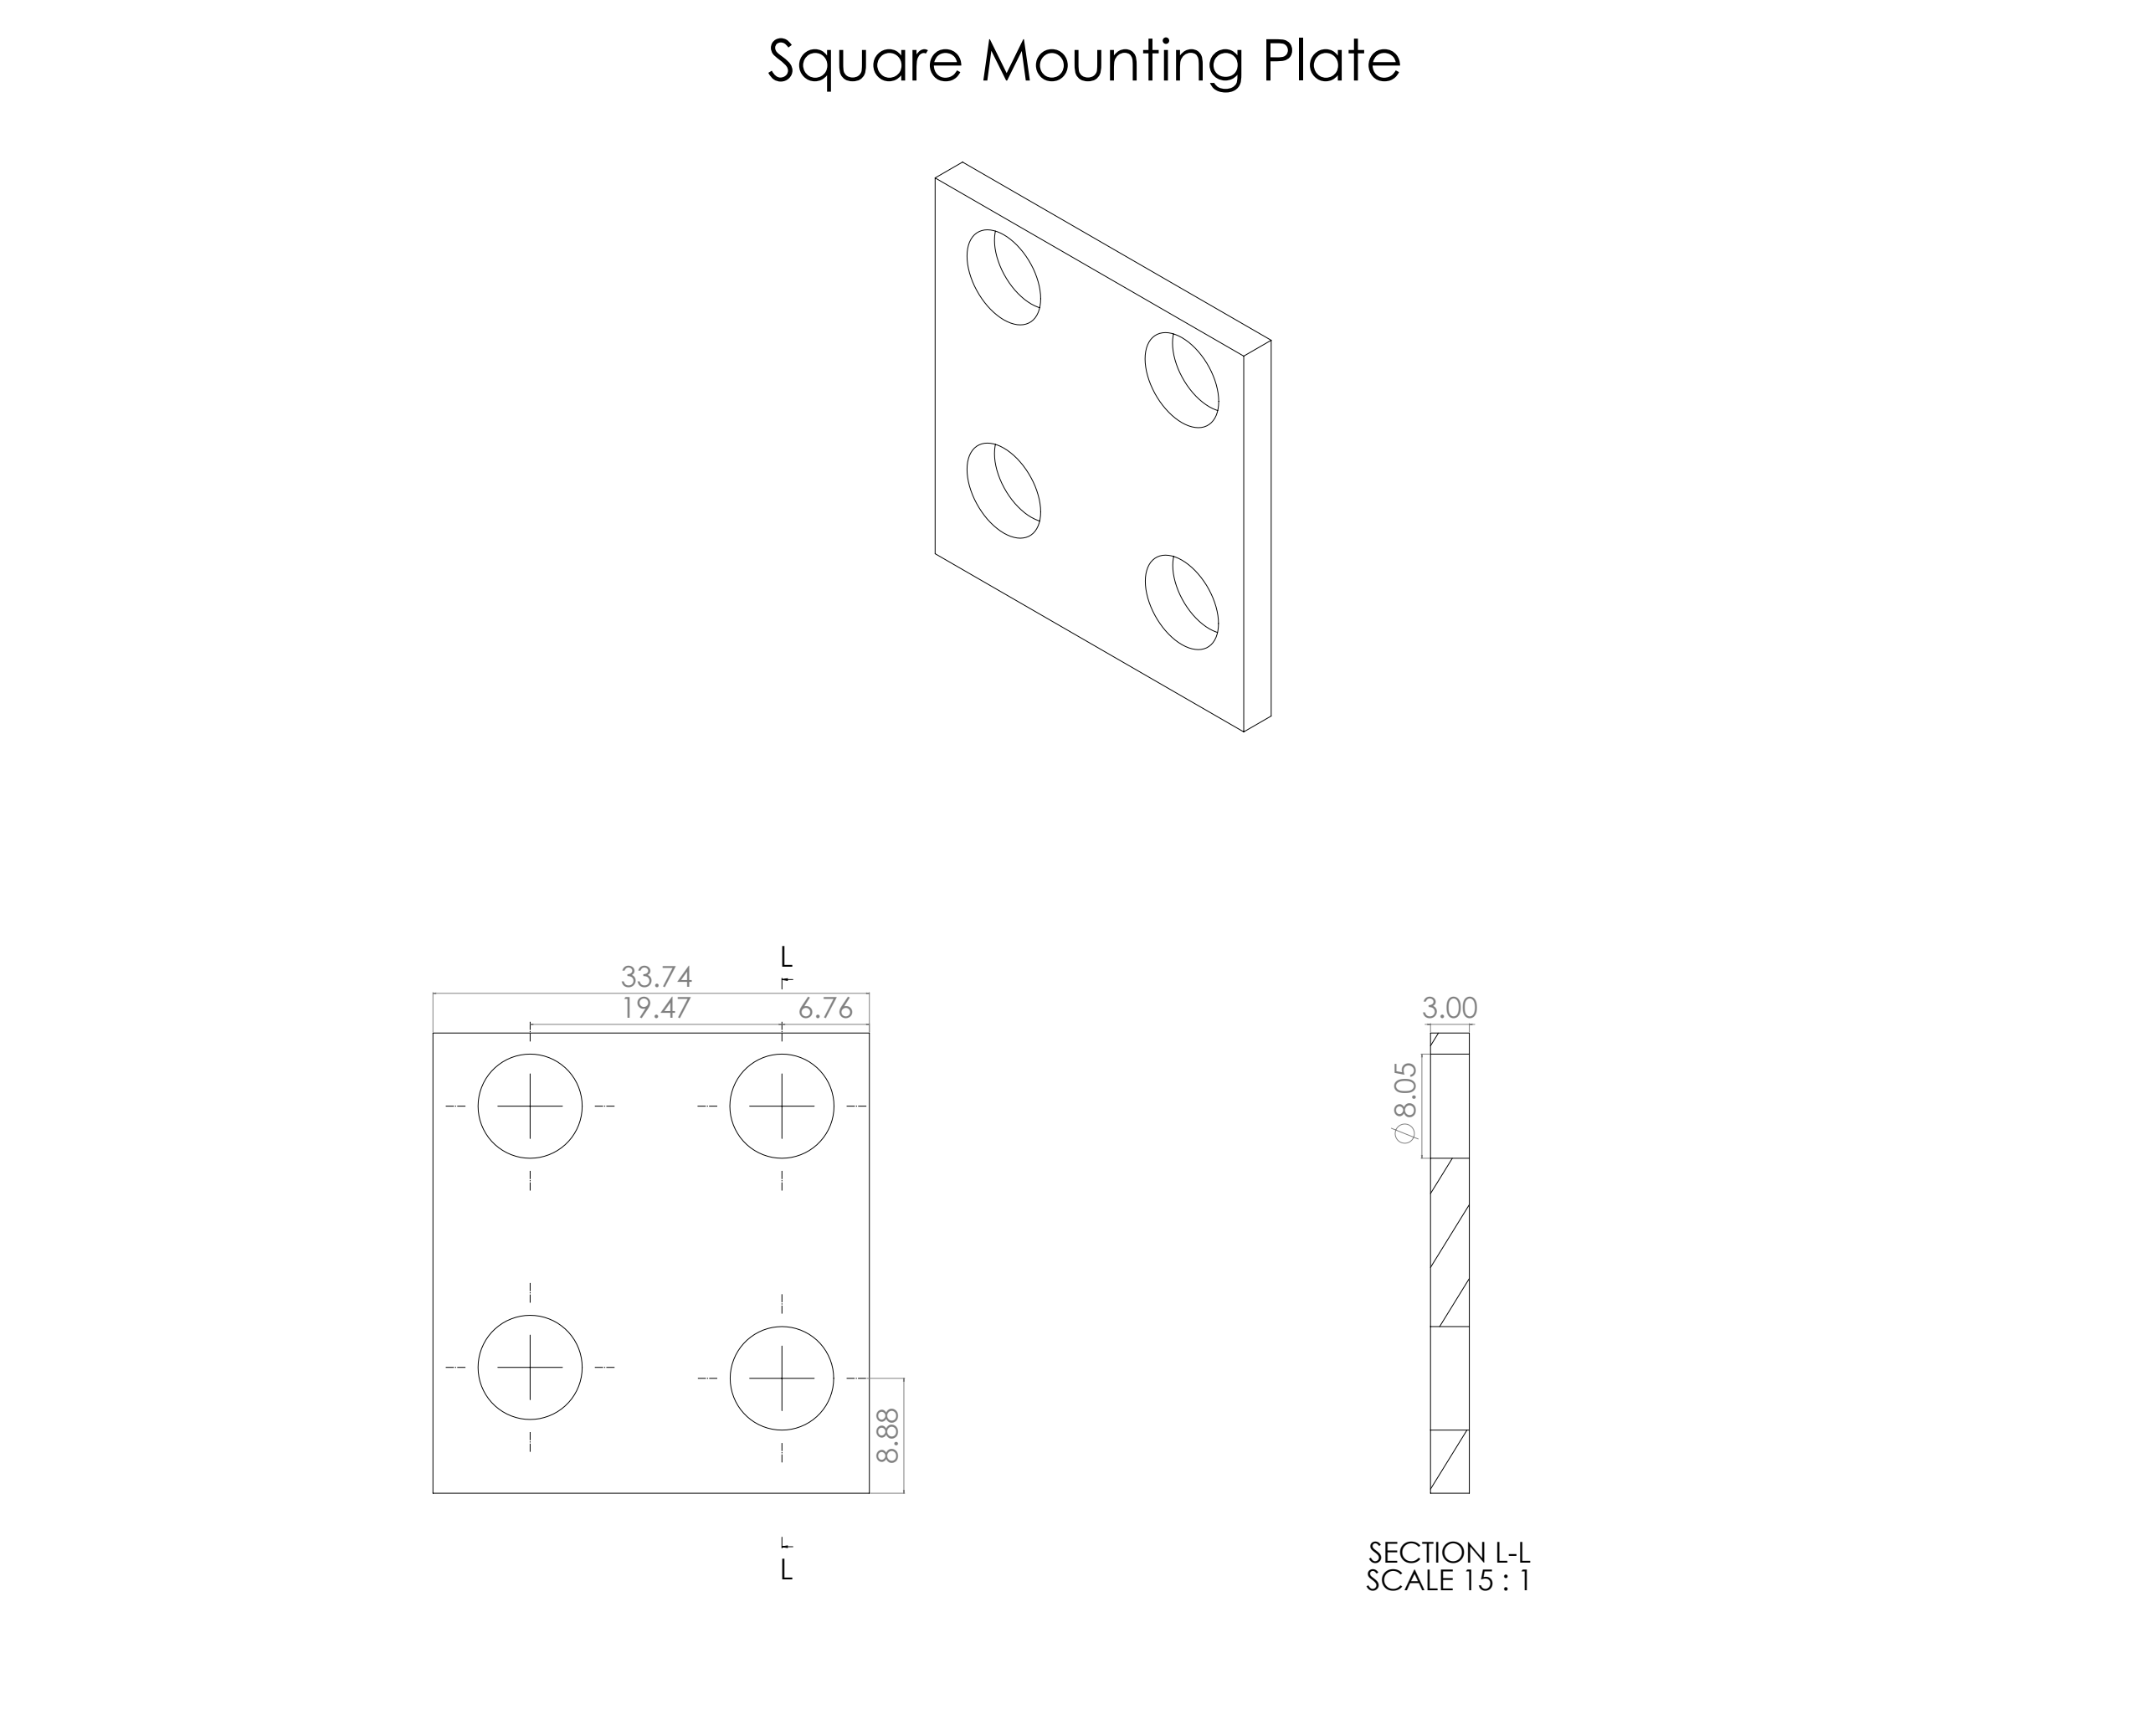
ISO-10303-21;
HEADER;
FILE_DESCRIPTION (('STEP AP214'),
    '1' );
FILE_NAME ('Square Mounting Plate.step',
    '2026-10-25T20:52:49',
    ( '' ),
    ( '' ),
    'SwSTEP 2.0',
    'SolidWorks 2025',
    '' );
FILE_SCHEMA (( 'AUTOMOTIVE_DESIGN' ));
ENDSEC;

DATA;
#8=AXIS2_PLACEMENT_3D ( 'NONE', #62573, #33196, #12356 ) ;
#139=DIRECTION ( 'NONE',  ( -0.000000000000000000, -0.000000000000000000, -1.000000000000000000 ) ) ;
#353=CARTESIAN_POINT ( 'NONE',  ( 184.7149167944524493, -12.49482340714361506, 10.00000000000000000 ) ) ;
#408=ORIENTED_EDGE ( 'NONE', *, *, #36940, .T. ) ;
#447=ADVANCED_FACE ( 'NONE', ( #62233, #49878, #84920, #20557, #27656 ), #19601, .F. ) ;
#551=CIRCLE ( 'NONE', #48930, 4.025000000000000355 ) ;
#864=UNCERTAINTY_MEASURE_WITH_UNIT (LENGTH_MEASURE( 1.000000000000000082E-05 ), #46095, 'distance_accuracy_value', 'NONE');
#1344=LINE ( 'NONE', #84136, #2329 ) ;
#1911=VERTEX_POINT ( 'NONE', #48237 ) ;
#1925=DIRECTION ( 'NONE',  ( 1.000000000000000000, 0.000000000000000000, 0.000000000000000000 ) ) ;
#2019=AXIS2_PLACEMENT_3D ( 'NONE', #11166, #32490, #12101 ) ;
#2104=VECTOR ( 'NONE', #19329, 1000.000000000000000 ) ;
#2329=VECTOR ( 'NONE', #75642, 1000.000000000000000 ) ;
#2393=ORIENTED_EDGE ( 'NONE', *, *, #76002, .F. ) ;
#2730=LINE ( 'NONE', #22180, #9659 ) ;
#2962=ORIENTED_EDGE ( 'NONE', *, *, #45806, .T. ) ;
#2974=ORIENTED_EDGE ( 'NONE', *, *, #32590, .F. ) ;
#3119=EDGE_CURVE ( 'NONE', #68047, #25647, #2730, .T. ) ;
#3129=PLANE ( 'NONE',  #2019 ) ;
#3367=ADVANCED_FACE ( 'NONE', ( #32552 ), #90725, .F. ) ;
#3593=DIRECTION ( 'NONE',  ( 0.000000000000000000, -1.000000000000000000, 0.000000000000000000 ) ) ;
#3609=DIRECTION ( 'NONE',  ( -0.000000000000000000, 1.000000000000000000, -0.000000000000000000 ) ) ;
#3701=ORIENTED_EDGE ( 'NONE', *, *, #20481, .F. ) ;
#4241=ORIENTED_EDGE ( 'NONE', *, *, #72732, .F. ) ;
#4407=CARTESIAN_POINT ( 'NONE',  ( 157.7374095173865385, 14.19731191252289015, 10.00000000000000000 ) ) ;
#4431=CARTESIAN_POINT ( 'NONE',  ( 157.7374095173865385, -21.37379927922774314, 13.00000000000000178 ) ) ;
#4459=CARTESIAN_POINT ( 'NONE',  ( 0.000000000000000000, 0.000000000000000000, 13.00000000000000178 ) ) ;
#4865=CARTESIAN_POINT ( 'NONE',  ( 165.2494399300530290, 8.542400036368780647, 13.00000000000000178 ) ) ;
#5292=AXIS2_PLACEMENT_3D ( 'NONE', #52984, #39682, #88956 ) ;
#5545=DIRECTION ( 'NONE',  ( -0.000000000000000000, -0.000000000000000000, -1.000000000000000000 ) ) ;
#5566=DIRECTION ( 'NONE',  ( 1.000000000000000000, 0.000000000000000000, 0.000000000000000000 ) ) ;
#5653=DIRECTION ( 'NONE',  ( 0.000000000000000000, 0.000000000000000000, 1.000000000000000000 ) ) ;
#5825=VECTOR ( 'NONE', #37864, 1000.000000000000000 ) ;
#6003=CYLINDRICAL_SURFACE ( 'NONE', #90095, 4.025000000000000355 ) ;
#6032=EDGE_CURVE ( 'NONE', #1911, #61737, #79312, .T. ) ;
#6390=CARTESIAN_POINT ( 'NONE',  ( 184.7149167944524493, 8.542400036368780647, 13.00000000000000178 ) ) ;
#6471=FACE_OUTER_BOUND ( 'NONE', #34561, .T. ) ;
#6537=DIRECTION ( 'NONE',  ( 0.000000000000000000, 0.000000000000000000, 1.000000000000000000 ) ) ;
#6539=CARTESIAN_POINT ( 'NONE',  ( 188.7399167944524550, 8.542400036368780647, 10.00000000000000000 ) ) ;
#6644=CIRCLE ( 'NONE', #42844, 4.025000000000000355 ) ;
#6791=ORIENTED_EDGE ( 'NONE', *, *, #15024, .T. ) ;
#6965=CARTESIAN_POINT ( 'NONE',  ( 184.7149167944524493, -12.49482340714361506, 13.00000000000000178 ) ) ;
#7630=DIRECTION ( 'NONE',  ( 0.000000000000000000, 0.000000000000000000, 1.000000000000000000 ) ) ;
#7706=ORIENTED_EDGE ( 'NONE', *, *, #10597, .T. ) ;
#7906=DIRECTION ( 'NONE',  ( 0.000000000000000000, -1.000000000000000000, 0.000000000000000000 ) ) ;
#8136=ADVANCED_FACE ( 'NONE', ( #24569 ), #18400, .F. ) ;
#8485=LINE ( 'NONE', #29817, #24717 ) ;
#8878=DIRECTION ( 'NONE',  ( 1.000000000000000000, 0.000000000000000000, 0.000000000000000000 ) ) ;
#9004=ORIENTED_EDGE ( 'NONE', *, *, #61815, .F. ) ;
#9377=PRODUCT_DEFINITION ( 'UNKNOWN', '', #37123, #92065 ) ;
#9659=VECTOR ( 'NONE', #77029, 1000.000000000000000 ) ;
#9802=DIRECTION ( 'NONE',  ( -1.000000000000000000, 0.000000000000000000, 0.000000000000000000 ) ) ;
#10162=ORIENTED_EDGE ( 'NONE', *, *, #76002, .T. ) ;
#10597=EDGE_CURVE ( 'NONE', #42154, #35472, #64044, .T. ) ;
#10869=SHAPE_DEFINITION_REPRESENTATION ( #16322, #67633 ) ;
#10909=ADVANCED_FACE ( 'NONE', ( #61387 ), #3129, .F. ) ;
#10927=DIRECTION ( 'NONE',  ( -0.000000000000000000, 1.000000000000000000, -0.000000000000000000 ) ) ;
#10938=ORIENTED_EDGE ( 'NONE', *, *, #71944, .T. ) ;
#11054=EDGE_CURVE ( 'NONE', #75279, #54193, #61836, .T. ) ;
#11126=ORIENTED_EDGE ( 'NONE', *, *, #61815, .T. ) ;
#11166=CARTESIAN_POINT ( 'NONE',  ( 191.4749582765727212, -21.37379927922774314, 13.00000000000000178 ) ) ;
#11214=ORIENTED_EDGE ( 'NONE', *, *, #3119, .F. ) ;
#11227=DIRECTION ( 'NONE',  ( -1.000000000000000000, 0.000000000000000000, 0.000000000000000000 ) ) ;
#11260=EDGE_CURVE ( 'NONE', #35472, #42154, #551, .T. ) ;
#12032=DIRECTION ( 'NONE',  ( -0.000000000000000000, 0.000000000000000000, -1.000000000000000000 ) ) ;
#12093=CARTESIAN_POINT ( 'NONE',  ( 157.7374095173865385, 14.19731191252289015, 13.00000000000000178 ) ) ;
#12101=DIRECTION ( 'NONE',  ( 0.000000000000000000, 0.000000000000000000, 1.000000000000000000 ) ) ;
#12158=DIRECTION ( 'NONE',  ( 0.000000000000000000, 0.000000000000000000, 1.000000000000000000 ) ) ;
#12159=CARTESIAN_POINT ( 'NONE',  ( 165.2494399300530290, -11.64849832608277325, 13.00000000000000178 ) ) ;
#12356=DIRECTION ( 'NONE',  ( 1.000000000000000000, 0.000000000000000000, 0.000000000000000000 ) ) ;
#12553=EDGE_CURVE ( 'NONE', #60279, #70988, #6644, .T. ) ;
#12633=VECTOR ( 'NONE', #3593, 1000.000000000000000 ) ;
#12712=CARTESIAN_POINT ( 'NONE',  ( 165.2494399300530290, 8.542400036368780647, 10.00000000000000000 ) ) ;
#12714=CARTESIAN_POINT ( 'NONE',  ( 161.2244399300530233, 8.542400036368780647, 13.00000000000000178 ) ) ;
#12853=ORIENTED_EDGE ( 'NONE', *, *, #17274, .F. ) ;
#13234=CARTESIAN_POINT ( 'NONE',  ( 157.7374095173865385, 14.19731191252289015, 13.00000000000000178 ) ) ;
#13610=DIRECTION ( 'NONE',  ( -0.000000000000000000, -0.000000000000000000, -1.000000000000000000 ) ) ;
#13683=VERTEX_POINT ( 'NONE', #44001 ) ;
#13955=ORIENTED_EDGE ( 'NONE', *, *, #89206, .T. ) ;
#13997=AXIS2_PLACEMENT_3D ( 'NONE', #6390, #21057, #20601 ) ;
#14168=CARTESIAN_POINT ( 'NONE',  ( 184.7149167944524493, 8.542400036368780647, 10.00000000000000000 ) ) ;
#14370=VERTEX_POINT ( 'NONE', #44472 ) ;
#15012=LINE ( 'NONE', #34924, #23160 ) ;
#15024=EDGE_CURVE ( 'NONE', #13683, #26669, #33933, .T. ) ;
#15028=DIRECTION ( 'NONE',  ( 0.000000000000000000, 0.000000000000000000, 1.000000000000000000 ) ) ;
#15052=CARTESIAN_POINT ( 'NONE',  ( 165.2494399300530290, -11.64849832608277325, 13.00000000000000178 ) ) ;
#15135=LINE ( 'NONE', #48894, #73055 ) ;
#15206=AXIS2_PLACEMENT_3D ( 'NONE', #88270, #45167, #75471 ) ;
#15346=( GEOMETRIC_REPRESENTATION_CONTEXT ( 3 ) GLOBAL_UNCERTAINTY_ASSIGNED_CONTEXT ( ( #864 ) ) GLOBAL_UNIT_ASSIGNED_CONTEXT ( ( #46095, #75000, #22926 ) ) REPRESENTATION_CONTEXT ( 'NONE', 'WORKASPACE' ) );
#15365=CYLINDRICAL_SURFACE ( 'NONE', #84868, 4.000000000000003553 ) ;
#15479=DIRECTION ( 'NONE',  ( 1.000000000000000000, 0.000000000000000000, 0.000000000000000000 ) ) ;
#15510=DIRECTION ( 'NONE',  ( -0.000000000000000000, -0.000000000000000000, -1.000000000000000000 ) ) ;
#15530=AXIS2_PLACEMENT_3D ( 'NONE', #4865, #91002, #77306 ) ;
#15570=VECTOR ( 'NONE', #139, 1000.000000000000000 ) ;
#15605=AXIS2_PLACEMENT_3D ( 'NONE', #59729, #88571, #45946 ) ;
#15644=EDGE_CURVE ( 'NONE', #54449, #93705, #66778, .T. ) ;
#16173=EDGE_CURVE ( 'NONE', #25647, #60166, #23043, .T. ) ;
#16322=PRODUCT_DEFINITION_SHAPE ( 'NONE', 'NONE',  #9377 ) ;
#16414=CARTESIAN_POINT ( 'NONE',  ( 157.7374095173865385, 14.19731191252289015, 10.00000000000000000 ) ) ;
#16631=DIRECTION ( 'NONE',  ( 0.000000000000000000, 0.000000000000000000, 1.000000000000000000 ) ) ;
#16908=CARTESIAN_POINT ( 'NONE',  ( 191.4749582765727212, -21.37379927922774314, 10.00000000000000000 ) ) ;
#16910=DIRECTION ( 'NONE',  ( 1.000000000000000000, 0.000000000000000000, 0.000000000000000000 ) ) ;
#17031=AXIS2_PLACEMENT_3D ( 'NONE', #6965, #37671, #45697 ) ;
#17057=PRODUCT_CONTEXT ( 'NONE', #52342, 'mechanical' ) ;
#17230=APPLICATION_CONTEXT ( 'automotive_design' ) ;
#17233=FACE_OUTER_BOUND ( 'NONE', #64373, .T. ) ;
#17274=EDGE_CURVE ( 'NONE', #75279, #79924, #47612, .T. ) ;
#17796=PLANE ( 'NONE',  #80542 ) ;
#17808=CARTESIAN_POINT ( 'NONE',  ( 165.2494399300530290, 8.542400036368780647, 13.00000000000000178 ) ) ;
#18181=EDGE_LOOP ( 'NONE', ( #55024, #55045, #4241, #85295 ) ) ;
#18204=EDGE_CURVE ( 'NONE', #60166, #54193, #90447, .T. ) ;
#18373=STYLED_ITEM('',(#93738),#58100);
#18377=CARTESIAN_POINT ( 'NONE',  ( 161.2244399300530233, 8.542400036368780647, 13.00000000000000178 ) ) ;
#18400=CYLINDRICAL_SURFACE ( 'NONE', #5292, 4.025000000000000355 ) ;
#18683=ORIENTED_EDGE ( 'NONE', *, *, #91573, .F. ) ;
#18731=FACE_BOUND ( 'NONE', #71920, .T. ) ;
#18940=AXIS2_PLACEMENT_3D ( 'NONE', #90959, #40773, #33703 ) ;
#19058=VERTEX_POINT ( 'NONE', #55447 ) ;
#19329=DIRECTION ( 'NONE',  ( -0.000000000000000000, -0.000000000000000000, -1.000000000000000000 ) ) ;
#19436=DIRECTION ( 'NONE',  ( -0.000000000000000000, -0.000000000000000000, -1.000000000000000000 ) ) ;
#19601=PLANE ( 'NONE',  #64162 ) ;
#19841=DIRECTION ( 'NONE',  ( -0.000000000000000000, 0.000000000000000000, -1.000000000000000000 ) ) ;
#20063=AXIS2_PLACEMENT_3D ( 'NONE', #71362, #56703, #5566 ) ;
#20449=CLOSED_SHELL ( 'NONE', ( #27401, #8136, #58097, #83433, #447, #23737, #3367, #41920, #88676, #10909, #93028, #88549, #21965, #23016 ) ) ;
#20454=ORIENTED_EDGE ( 'NONE', *, *, #88734, .F. ) ;
#20481=EDGE_CURVE ( 'NONE', #26669, #13683, #83518, .T. ) ;
#20511=CARTESIAN_POINT ( 'NONE',  ( 191.4749582765727212, -21.37379927922774314, 13.00000000000000178 ) ) ;
#20557=FACE_BOUND ( 'NONE', #43970, .T. ) ;
#20601=DIRECTION ( 'NONE',  ( -1.000000000000000000, 0.000000000000000000, 0.000000000000000000 ) ) ;
#21057=DIRECTION ( 'NONE',  ( -0.000000000000000000, -0.000000000000000000, -1.000000000000000000 ) ) ;
#21296=CIRCLE ( 'NONE', #15206, 4.025000000000000355 ) ;
#21478=ORIENTED_EDGE ( 'NONE', *, *, #26156, .F. ) ;
#21481=EDGE_LOOP ( 'NONE', ( #73742, #54532, #408, #40993 ) ) ;
#21520=FACE_OUTER_BOUND ( 'NONE', #59218, .T. ) ;
#21649=VECTOR ( 'NONE', #25477, 1000.000000000000000 ) ;
#21965=ADVANCED_FACE ( 'NONE', ( #21520 ), #73117, .F. ) ;
#22003=CIRCLE ( 'NONE', #56760, 4.025000000000000355 ) ;
#22180=CARTESIAN_POINT ( 'NONE',  ( 157.7374095173865385, 14.19731191252289015, 13.00000000000000178 ) ) ;
#22629=DIRECTION ( 'NONE',  ( 0.000000000000000000, 0.000000000000000000, 1.000000000000000000 ) ) ;
#22699=VECTOR ( 'NONE', #43051, 1000.000000000000000 ) ;
#22926=( NAMED_UNIT ( * ) SI_UNIT ( $, .STERADIAN. ) SOLID_ANGLE_UNIT ( ) );
#23016=ADVANCED_FACE ( 'NONE', ( #77785 ), #48403, .F. ) ;
#23025=CIRCLE ( 'NONE', #79013, 4.025000000000000355 ) ;
#23029=VECTOR ( 'NONE', #40726, 1000.000000000000000 ) ;
#23043=LINE ( 'NONE', #16414, #63840 ) ;
#23160=VECTOR ( 'NONE', #56730, 1000.000000000000000 ) ;
#23554=FACE_OUTER_BOUND ( 'NONE', #33852, .T. ) ;
#23680=CARTESIAN_POINT ( 'NONE',  ( 161.2244399300530233, -11.64849832608277325, 13.00000000000000178 ) ) ;
#23737=ADVANCED_FACE ( 'NONE', ( #18731, #41416, #47592, #55191, #68451 ), #17796, .T. ) ;
#23972=DIRECTION ( 'NONE',  ( 0.000000000000000000, 0.000000000000000000, 1.000000000000000000 ) ) ;
#24007=DIRECTION ( 'NONE',  ( 0.000000000000000000, 0.000000000000000000, 1.000000000000000000 ) ) ;
#24051=DIRECTION ( 'NONE',  ( 0.000000000000000000, 0.000000000000000000, 1.000000000000000000 ) ) ;
#24063=ORIENTED_EDGE ( 'NONE', *, *, #83965, .F. ) ;
#24181=CARTESIAN_POINT ( 'NONE',  ( 191.4749582765727212, 14.19731191252289015, 13.00000000000000178 ) ) ;
#24569=FACE_OUTER_BOUND ( 'NONE', #90079, .T. ) ;
#24717=VECTOR ( 'NONE', #77795, 1000.000000000000000 ) ;
#24915=CARTESIAN_POINT ( 'NONE',  ( 191.4749582765727212, -21.37379927922774314, 13.00000000000000178 ) ) ;
#25102=ORIENTED_EDGE ( 'NONE', *, *, #11054, .F. ) ;
#25477=DIRECTION ( 'NONE',  ( -0.000000000000000000, -0.000000000000000000, -1.000000000000000000 ) ) ;
#25493=LINE ( 'NONE', #12714, #2104 ) ;
#25592=LINE ( 'NONE', #54475, #91229 ) ;
#25647=VERTEX_POINT ( 'NONE', #4407 ) ;
#26156=EDGE_CURVE ( 'NONE', #78471, #75279, #15135, .T. ) ;
#26218=PRODUCT ( 'Square Mounting Plate', 'Square Mounting Plate', '', ( #17057 ) ) ;
#26330=EDGE_CURVE ( 'NONE', #79924, #68047, #8485, .T. ) ;
#26438=DIRECTION ( 'NONE',  ( 1.000000000000000000, 0.000000000000000000, 0.000000000000000000 ) ) ;
#26669=VERTEX_POINT ( 'NONE', #31668 ) ;
#27401=ADVANCED_FACE ( 'NONE', ( #82659 ), #52386, .F. ) ;
#27656=FACE_BOUND ( 'NONE', #56348, .T. ) ;
#27692=EDGE_LOOP ( 'NONE', ( #13955, #11214, #57944, #32676 ) ) ;
#27825=LINE ( 'NONE', #35844, #56523 ) ;
#27840=CARTESIAN_POINT ( 'NONE',  ( 161.2244399300530233, -11.64849832608277325, 10.00000000000000000 ) ) ;
#28163=CIRCLE ( 'NONE', #62975, 4.025000000000000355 ) ;
#28563=ORIENTED_EDGE ( 'NONE', *, *, #18204, .F. ) ;
#29388=EDGE_CURVE ( 'NONE', #54193, #19058, #75803, .T. ) ;
#29408=AXIS2_PLACEMENT_3D ( 'NONE', #90791, #62914, #26438 ) ;
#29498=ADVANCED_BREP_SHAPE_REPRESENTATION ( '', ( #58100, #18940 ), #56754 ) ;
#29762=ORIENTED_EDGE ( 'NONE', *, *, #26156, .T. ) ;
#29817=CARTESIAN_POINT ( 'NONE',  ( 191.4749582765727212, 14.19731191252289015, 13.00000000000000178 ) ) ;
#30553=ORIENTED_EDGE ( 'NONE', *, *, #18204, .T. ) ;
#30984=DIRECTION ( 'NONE',  ( -1.000000000000000000, 0.000000000000000000, 0.000000000000000000 ) ) ;
#31024=CARTESIAN_POINT ( 'NONE',  ( 161.2244399300530233, 8.542400036368780647, 10.00000000000000000 ) ) ;
#31087=DIRECTION ( 'NONE',  ( -0.000000000000000000, -0.000000000000000000, -1.000000000000000000 ) ) ;
#31668=CARTESIAN_POINT ( 'NONE',  ( 188.7149167944524493, -12.49482340714361506, 13.00000000000000178 ) ) ;
#32179=LINE ( 'NONE', #66768, #5825 ) ;
#32490=DIRECTION ( 'NONE',  ( 0.000000000000000000, 1.000000000000000000, -0.000000000000000000 ) ) ;
#32552=FACE_OUTER_BOUND ( 'NONE', #87279, .T. ) ;
#32590=EDGE_CURVE ( 'NONE', #79924, #19058, #57410, .T. ) ;
#32601=CARTESIAN_POINT ( 'NONE',  ( 191.4749582765727212, 14.19731191252289015, 13.00000000000000178 ) ) ;
#32676=ORIENTED_EDGE ( 'NONE', *, *, #32590, .T. ) ;
#33196=DIRECTION ( 'NONE',  ( 0.000000000000000000, 0.000000000000000000, 1.000000000000000000 ) ) ;
#33237=ORIENTED_EDGE ( 'NONE', *, *, #88734, .T. ) ;
#33703=DIRECTION ( 'NONE',  ( 1.000000000000000000, 0.000000000000000000, 0.000000000000000000 ) ) ;
#33711=CIRCLE ( 'NONE', #20063, 4.025000000000000355 ) ;
#33852=EDGE_LOOP ( 'NONE', ( #55744, #55923, #54648, #81093 ) ) ;
#33933=CIRCLE ( 'NONE', #29408, 4.000000000000003553 ) ;
#33939=AXIS2_PLACEMENT_3D ( 'NONE', #353, #15028, #43887 ) ;
#34528=FACE_OUTER_BOUND ( 'NONE', #21481, .T. ) ;
#34561=EDGE_LOOP ( 'NONE', ( #41948, #48478, #58414, #44534 ) ) ;
#34726=ORIENTED_EDGE ( 'NONE', *, *, #39657, .T. ) ;
#34779=ORIENTED_EDGE ( 'NONE', *, *, #51522, .T. ) ;
#34924=CARTESIAN_POINT ( 'NONE',  ( 169.2744399300530347, 8.542400036368780647, 13.00000000000000178 ) ) ;
#35006=LINE ( 'NONE', #77637, #22699 ) ;
#35018=AXIS2_PLACEMENT_3D ( 'NONE', #12712, #6537, #65245 ) ;
#35472=VERTEX_POINT ( 'NONE', #48415 ) ;
#35844=CARTESIAN_POINT ( 'NONE',  ( 180.6899167944524436, 8.542400036368780647, 13.00000000000000178 ) ) ;
#36042=EDGE_LOOP ( 'NONE', ( #34779, #43065, #77126, #64284 ) ) ;
#36581=LINE ( 'NONE', #71190, #15570 ) ;
#36781=CARTESIAN_POINT ( 'NONE',  ( 157.7374095173865385, -21.37379927922774314, 13.00000000000000178 ) ) ;
#36863=AXIS2_PLACEMENT_3D ( 'NONE', #88858, #24007, #16910 ) ;
#36940=EDGE_CURVE ( 'NONE', #13683, #61737, #25592, .T. ) ;
#37123=PRODUCT_DEFINITION_FORMATION_WITH_SPECIFIED_SOURCE ( 'ANY', '', #26218, .NOT_KNOWN. ) ;
#37671=DIRECTION ( 'NONE',  ( 0.000000000000000000, 0.000000000000000000, 1.000000000000000000 ) ) ;
#37864=DIRECTION ( 'NONE',  ( -0.000000000000000000, -0.000000000000000000, -1.000000000000000000 ) ) ;
#38735=EDGE_CURVE ( 'NONE', #70988, #54449, #25493, .T. ) ;
#39273=VERTEX_POINT ( 'NONE', #6539 ) ;
#39656=PLANE ( 'NONE',  #70119 ) ;
#39657=EDGE_CURVE ( 'NONE', #61737, #1911, #86848, .T. ) ;
#39682=DIRECTION ( 'NONE',  ( -0.000000000000000000, -0.000000000000000000, -1.000000000000000000 ) ) ;
#39846=CARTESIAN_POINT ( 'NONE',  ( 169.2744399300530347, 8.542400036368780647, 10.00000000000000000 ) ) ;
#40592=DIRECTION ( 'NONE',  ( 0.000000000000000000, -1.000000000000000000, 0.000000000000000000 ) ) ;
#40726=DIRECTION ( 'NONE',  ( 1.000000000000000000, -0.000000000000000000, -0.000000000000000000 ) ) ;
#40773=DIRECTION ( 'NONE',  ( 0.000000000000000000, 0.000000000000000000, 1.000000000000000000 ) ) ;
#40993=ORIENTED_EDGE ( 'NONE', *, *, #6032, .F. ) ;
#41416=FACE_BOUND ( 'NONE', #43459, .T. ) ;
#41475=ORIENTED_EDGE ( 'NONE', *, *, #89206, .F. ) ;
#41567=EDGE_CURVE ( 'NONE', #45901, #42154, #90323, .T. ) ;
#41920=ADVANCED_FACE ( 'NONE', ( #62900 ), #39656, .F. ) ;
#41948=ORIENTED_EDGE ( 'NONE', *, *, #78922, .F. ) ;
#42154=VERTEX_POINT ( 'NONE', #27840 ) ;
#42562=MECHANICAL_DESIGN_GEOMETRIC_PRESENTATION_REPRESENTATION('',(#18373),#15346);
#42844=AXIS2_PLACEMENT_3D ( 'NONE', #53556, #16631, #89983 ) ;
#43051=DIRECTION ( 'NONE',  ( -0.000000000000000000, -0.000000000000000000, -1.000000000000000000 ) ) ;
#43065=ORIENTED_EDGE ( 'NONE', *, *, #71361, .T. ) ;
#43288=EDGE_LOOP ( 'NONE', ( #54099, #11126 ) ) ;
#43459=EDGE_LOOP ( 'NONE', ( #7706, #69578 ) ) ;
#43871=LINE ( 'NONE', #36781, #54989 ) ;
#43887=DIRECTION ( 'NONE',  ( 1.000000000000000000, 0.000000000000000000, 0.000000000000000000 ) ) ;
#43970=EDGE_LOOP ( 'NONE', ( #73348, #67827 ) ) ;
#43998=DIRECTION ( 'NONE',  ( 1.000000000000000000, -0.000000000000000000, -0.000000000000000000 ) ) ;
#44001=CARTESIAN_POINT ( 'NONE',  ( 180.7149167944524493, -12.49482340714361506, 13.00000000000000178 ) ) ;
#44128=VERTEX_POINT ( 'NONE', #49507 ) ;
#44472=CARTESIAN_POINT ( 'NONE',  ( 188.7399167944524550, 8.542400036368780647, 13.00000000000000178 ) ) ;
#44534=ORIENTED_EDGE ( 'NONE', *, *, #11260, .F. ) ;
#45167=DIRECTION ( 'NONE',  ( 0.000000000000000000, 0.000000000000000000, 1.000000000000000000 ) ) ;
#45353=ORIENTED_EDGE ( 'NONE', *, *, #91573, .T. ) ;
#45697=DIRECTION ( 'NONE',  ( 1.000000000000000000, 0.000000000000000000, 0.000000000000000000 ) ) ;
#45768=CYLINDRICAL_SURFACE ( 'NONE', #61072, 4.025000000000000355 ) ;
#45806=EDGE_CURVE ( 'NONE', #26669, #1911, #32179, .T. ) ;
#45901=VERTEX_POINT ( 'NONE', #23680 ) ;
#45917=ORIENTED_EDGE ( 'NONE', *, *, #62258, .T. ) ;
#45946=DIRECTION ( 'NONE',  ( 1.000000000000000000, 0.000000000000000000, 0.000000000000000000 ) ) ;
#46095=( LENGTH_UNIT ( ) NAMED_UNIT ( * ) SI_UNIT ( .MILLI., .METRE. ) );
#46335=CARTESIAN_POINT ( 'NONE',  ( 157.7374095173865385, -21.37379927922774314, 10.00000000000000000 ) ) ;
#46649=DIRECTION ( 'NONE',  ( -1.000000000000000000, 0.000000000000000000, 0.000000000000000000 ) ) ;
#46661=DIRECTION ( 'NONE',  ( -0.000000000000000000, -0.000000000000000000, -1.000000000000000000 ) ) ;
#46696=ORIENTED_EDGE ( 'NONE', *, *, #29388, .F. ) ;
#47592=FACE_OUTER_BOUND ( 'NONE', #54104, .T. ) ;
#47612=LINE ( 'NONE', #68005, #85014 ) ;
#47652=AXIS2_PLACEMENT_3D ( 'NONE', #49197, #84694, #70528 ) ;
#48060=LINE ( 'NONE', #12093, #12633 ) ;
#48237=CARTESIAN_POINT ( 'NONE',  ( 188.7149167944524493, -12.49482340714361506, 10.00000000000000000 ) ) ;
#48403=CYLINDRICAL_SURFACE ( 'NONE', #15530, 4.025000000000000355 ) ;
#48415=CARTESIAN_POINT ( 'NONE',  ( 169.2744399300530347, -11.64849832608277325, 10.00000000000000000 ) ) ;
#48478=ORIENTED_EDGE ( 'NONE', *, *, #77975, .T. ) ;
#48894=CARTESIAN_POINT ( 'NONE',  ( 191.4749582765727212, -21.37379927922774314, 13.00000000000000178 ) ) ;
#48930=AXIS2_PLACEMENT_3D ( 'NONE', #63734, #58013, #72220 ) ;
#49017=VECTOR ( 'NONE', #53544, 1000.000000000000000 ) ;
#49171=EDGE_LOOP ( 'NONE', ( #34726, #73801 ) ) ;
#49197=CARTESIAN_POINT ( 'NONE',  ( 184.7149167944524493, -12.49482340714361506, 13.00000000000000178 ) ) ;
#49507=CARTESIAN_POINT ( 'NONE',  ( 180.6899167944524436, 8.542400036368780647, 13.00000000000000178 ) ) ;
#49644=EDGE_LOOP ( 'NONE', ( #30553, #25102, #21478, #10938 ) ) ;
#49878=FACE_BOUND ( 'NONE', #52581, .T. ) ;
#51413=CIRCLE ( 'NONE', #8, 4.025000000000000355 ) ;
#51522=EDGE_CURVE ( 'NONE', #70988, #60279, #51413, .T. ) ;
#51626=( NAMED_UNIT ( * ) PLANE_ANGLE_UNIT ( ) SI_UNIT ( $, .RADIAN. ) );
#52342=APPLICATION_CONTEXT ( 'automotive_design' ) ;
#52386=CYLINDRICAL_SURFACE ( 'NONE', #80483, 4.025000000000000355 ) ;
#52581=EDGE_LOOP ( 'NONE', ( #24063, #88414 ) ) ;
#52984=CARTESIAN_POINT ( 'NONE',  ( 184.7149167944524493, 8.542400036368780647, 13.00000000000000178 ) ) ;
#53275=ORIENTED_EDGE ( 'NONE', *, *, #39657, .F. ) ;
#53288=CARTESIAN_POINT ( 'NONE',  ( 157.7374095173865385, 14.19731191252289015, 13.00000000000000178 ) ) ;
#53544=DIRECTION ( 'NONE',  ( -0.000000000000000000, -0.000000000000000000, -1.000000000000000000 ) ) ;
#53556=CARTESIAN_POINT ( 'NONE',  ( 165.2494399300530290, 8.542400036368780647, 13.00000000000000178 ) ) ;
#53631=ORIENTED_EDGE ( 'NONE', *, *, #66872, .F. ) ;
#54099=ORIENTED_EDGE ( 'NONE', *, *, #15644, .T. ) ;
#54104=EDGE_LOOP ( 'NONE', ( #46696, #28563, #76477, #41475 ) ) ;
#54193=VERTEX_POINT ( 'NONE', #16908 ) ;
#54449=VERTEX_POINT ( 'NONE', #31024 ) ;
#54475=CARTESIAN_POINT ( 'NONE',  ( 180.7149167944524493, -12.49482340714361506, 13.00000000000000178 ) ) ;
#54532=ORIENTED_EDGE ( 'NONE', *, *, #20481, .T. ) ;
#54648=ORIENTED_EDGE ( 'NONE', *, *, #10597, .F. ) ;
#54989=VECTOR ( 'NONE', #31087, 1000.000000000000000 ) ;
#55024=ORIENTED_EDGE ( 'NONE', *, *, #16173, .T. ) ;
#55045=ORIENTED_EDGE ( 'NONE', *, *, #71944, .F. ) ;
#55191=FACE_BOUND ( 'NONE', #49171, .T. ) ;
#55447=CARTESIAN_POINT ( 'NONE',  ( 191.4749582765727212, 14.19731191252289015, 10.00000000000000000 ) ) ;
#55744=ORIENTED_EDGE ( 'NONE', *, *, #83965, .T. ) ;
#55839=CYLINDRICAL_SURFACE ( 'NONE', #47652, 4.000000000000003553 ) ;
#55923=ORIENTED_EDGE ( 'NONE', *, *, #78922, .T. ) ;
#56348=EDGE_LOOP ( 'NONE', ( #56806, #76708 ) ) ;
#56523=VECTOR ( 'NONE', #13610, 1000.000000000000000 ) ;
#56607=AXIS2_PLACEMENT_3D ( 'NONE', #65430, #7630, #1925 ) ;
#56703=DIRECTION ( 'NONE',  ( 0.000000000000000000, 0.000000000000000000, 1.000000000000000000 ) ) ;
#56730=DIRECTION ( 'NONE',  ( -0.000000000000000000, -0.000000000000000000, -1.000000000000000000 ) ) ;
#56754=( GEOMETRIC_REPRESENTATION_CONTEXT ( 3 ) GLOBAL_UNCERTAINTY_ASSIGNED_CONTEXT ( ( #57980 ) ) GLOBAL_UNIT_ASSIGNED_CONTEXT ( ( #65421, #51626, #74343 ) ) REPRESENTATION_CONTEXT ( 'NONE', 'WORKASPACE' ) );
#56760=AXIS2_PLACEMENT_3D ( 'NONE', #14168, #5653, #85177 ) ;
#56806=ORIENTED_EDGE ( 'NONE', *, *, #51522, .F. ) ;
#56975=CARTESIAN_POINT ( 'NONE',  ( 169.2744399300530347, -11.64849832608277325, 13.00000000000000178 ) ) ;
#57256=FACE_OUTER_BOUND ( 'NONE', #18181, .T. ) ;
#57410=LINE ( 'NONE', #24181, #49017 ) ;
#57944=ORIENTED_EDGE ( 'NONE', *, *, #26330, .F. ) ;
#57980=UNCERTAINTY_MEASURE_WITH_UNIT (LENGTH_MEASURE( 1.000000000000000082E-05 ), #65421, 'distance_accuracy_value', 'NONE');
#58013=DIRECTION ( 'NONE',  ( 0.000000000000000000, 0.000000000000000000, 1.000000000000000000 ) ) ;
#58097=ADVANCED_FACE ( 'NONE', ( #17233 ), #15365, .F. ) ;
#58100=MANIFOLD_SOLID_BREP ( 'Boss-Extrude20', #20449 ) ;
#58414=ORIENTED_EDGE ( 'NONE', *, *, #41567, .T. ) ;
#58767=ORIENTED_EDGE ( 'NONE', *, *, #36940, .F. ) ;
#58926=CARTESIAN_POINT ( 'NONE',  ( 184.7149167944524493, -12.49482340714361506, 13.00000000000000178 ) ) ;
#59122=CARTESIAN_POINT ( 'NONE',  ( 180.7149167944524493, -12.49482340714361506, 10.00000000000000000 ) ) ;
#59218=EDGE_LOOP ( 'NONE', ( #2393, #45917, #81571, #20454 ) ) ;
#59550=VERTEX_POINT ( 'NONE', #61611 ) ;
#59729=CARTESIAN_POINT ( 'NONE',  ( 184.7149167944524493, 8.542400036368780647, 13.00000000000000178 ) ) ;
#59984=CARTESIAN_POINT ( 'NONE',  ( 165.2494399300530290, -11.64849832608277325, 10.00000000000000000 ) ) ;
#60063=CARTESIAN_POINT ( 'NONE',  ( 165.2494399300530290, 8.542400036368780647, 10.00000000000000000 ) ) ;
#60166=VERTEX_POINT ( 'NONE', #46335 ) ;
#60279=VERTEX_POINT ( 'NONE', #83253 ) ;
#61072=AXIS2_PLACEMENT_3D ( 'NONE', #15052, #15510, #9802 ) ;
#61171=ORIENTED_EDGE ( 'NONE', *, *, #38735, .T. ) ;
#61387=FACE_OUTER_BOUND ( 'NONE', #49644, .T. ) ;
#61611=CARTESIAN_POINT ( 'NONE',  ( 180.6899167944524436, 8.542400036368780647, 10.00000000000000000 ) ) ;
#61737=VERTEX_POINT ( 'NONE', #59122 ) ;
#61815=EDGE_CURVE ( 'NONE', #93705, #54449, #23025, .T. ) ;
#61836=LINE ( 'NONE', #24915, #74610 ) ;
#62233=FACE_OUTER_BOUND ( 'NONE', #85988, .T. ) ;
#62258=EDGE_CURVE ( 'NONE', #14370, #44128, #33711, .T. ) ;
#62573=CARTESIAN_POINT ( 'NONE',  ( 165.2494399300530290, 8.542400036368780647, 13.00000000000000178 ) ) ;
#62900=FACE_OUTER_BOUND ( 'NONE', #27692, .T. ) ;
#62914=DIRECTION ( 'NONE',  ( 0.000000000000000000, 0.000000000000000000, 1.000000000000000000 ) ) ;
#62964=CARTESIAN_POINT ( 'NONE',  ( 184.7149167944524493, 8.542400036368780647, 10.00000000000000000 ) ) ;
#62975=AXIS2_PLACEMENT_3D ( 'NONE', #62964, #22629, #8878 ) ;
#63734=CARTESIAN_POINT ( 'NONE',  ( 165.2494399300530290, -11.64849832608277325, 10.00000000000000000 ) ) ;
#63840=VECTOR ( 'NONE', #7906, 1000.000000000000000 ) ;
#64044=CIRCLE ( 'NONE', #73135, 4.025000000000000355 ) ;
#64162=AXIS2_PLACEMENT_3D ( 'NONE', #4459, #12032, #92488 ) ;
#64284=ORIENTED_EDGE ( 'NONE', *, *, #38735, .F. ) ;
#64303=ORIENTED_EDGE ( 'NONE', *, *, #17274, .T. ) ;
#64373=EDGE_LOOP ( 'NONE', ( #6791, #2962, #53275, #58767 ) ) ;
#64488=EDGE_CURVE ( 'NONE', #44128, #14370, #73057, .T. ) ;
#64967=ORIENTED_EDGE ( 'NONE', *, *, #26330, .T. ) ;
#65245=DIRECTION ( 'NONE',  ( 1.000000000000000000, 0.000000000000000000, 0.000000000000000000 ) ) ;
#65421=( LENGTH_UNIT ( ) NAMED_UNIT ( * ) SI_UNIT ( .MILLI., .METRE. ) );
#65430=CARTESIAN_POINT ( 'NONE',  ( 184.7149167944524493, -12.49482340714361506, 10.00000000000000000 ) ) ;
#66768=CARTESIAN_POINT ( 'NONE',  ( 188.7149167944524493, -12.49482340714361506, 13.00000000000000178 ) ) ;
#66778=CIRCLE ( 'NONE', #35018, 4.025000000000000355 ) ;
#66853=ORIENTED_EDGE ( 'NONE', *, *, #11054, .T. ) ;
#66872=EDGE_CURVE ( 'NONE', #44128, #59550, #27825, .T. ) ;
#67578=ORIENTED_EDGE ( 'NONE', *, *, #29388, .T. ) ;
#67633=SHAPE_REPRESENTATION ( 'Square Mounting Plate', ( #18940 ), #56754 ) ;
#67827=ORIENTED_EDGE ( 'NONE', *, *, #62258, .F. ) ;
#68005=CARTESIAN_POINT ( 'NONE',  ( 191.4749582765727212, 14.19731191252289015, 13.00000000000000178 ) ) ;
#68047=VERTEX_POINT ( 'NONE', #53288 ) ;
#68451=FACE_BOUND ( 'NONE', #43288, .T. ) ;
#68716=CARTESIAN_POINT ( 'NONE',  ( 191.4749582765727212, -21.37379927922774314, 10.00000000000000000 ) ) ;
#69578=ORIENTED_EDGE ( 'NONE', *, *, #11260, .T. ) ;
#70119=AXIS2_PLACEMENT_3D ( 'NONE', #32601, #40592, #84629 ) ;
#70528=DIRECTION ( 'NONE',  ( -1.000000000000000000, 0.000000000000000000, 0.000000000000000000 ) ) ;
#70988=VERTEX_POINT ( 'NONE', #18377 ) ;
#71190=CARTESIAN_POINT ( 'NONE',  ( 169.2744399300530347, -11.64849832608277325, 13.00000000000000178 ) ) ;
#71361=EDGE_CURVE ( 'NONE', #60279, #93705, #15012, .T. ) ;
#71362=CARTESIAN_POINT ( 'NONE',  ( 184.7149167944524493, 8.542400036368780647, 13.00000000000000178 ) ) ;
#71920=EDGE_LOOP ( 'NONE', ( #45353, #33237 ) ) ;
#71944=EDGE_CURVE ( 'NONE', #78471, #60166, #43871, .T. ) ;
#72220=DIRECTION ( 'NONE',  ( 1.000000000000000000, 0.000000000000000000, 0.000000000000000000 ) ) ;
#72376=EDGE_LOOP ( 'NONE', ( #81238, #3701 ) ) ;
#72732=EDGE_CURVE ( 'NONE', #68047, #78471, #48060, .T. ) ;
#73055=VECTOR ( 'NONE', #43998, 1000.000000000000000 ) ;
#73057=CIRCLE ( 'NONE', #15605, 4.025000000000000355 ) ;
#73117=CYLINDRICAL_SURFACE ( 'NONE', #13997, 4.025000000000000355 ) ;
#73135=AXIS2_PLACEMENT_3D ( 'NONE', #59984, #23972, #15479 ) ;
#73348=ORIENTED_EDGE ( 'NONE', *, *, #64488, .F. ) ;
#73456=ORIENTED_EDGE ( 'NONE', *, *, #64488, .T. ) ;
#73742=ORIENTED_EDGE ( 'NONE', *, *, #45806, .F. ) ;
#73787=DIRECTION ( 'NONE',  ( 1.000000000000000000, 0.000000000000000000, 0.000000000000000000 ) ) ;
#73801=ORIENTED_EDGE ( 'NONE', *, *, #6032, .T. ) ;
#74343=( NAMED_UNIT ( * ) SI_UNIT ( $, .STERADIAN. ) SOLID_ANGLE_UNIT ( ) );
#74610=VECTOR ( 'NONE', #82660, 1000.000000000000000 ) ;
#74614=ORIENTED_EDGE ( 'NONE', *, *, #72732, .T. ) ;
#75000=( NAMED_UNIT ( * ) PLANE_ANGLE_UNIT ( ) SI_UNIT ( $, .RADIAN. ) );
#75154=VERTEX_POINT ( 'NONE', #56975 ) ;
#75279=VERTEX_POINT ( 'NONE', #20511 ) ;
#75345=CARTESIAN_POINT ( 'NONE',  ( 191.4749582765727212, 14.19731191252289015, 10.00000000000000000 ) ) ;
#75471=DIRECTION ( 'NONE',  ( 1.000000000000000000, 0.000000000000000000, 0.000000000000000000 ) ) ;
#75565=DIRECTION ( 'NONE',  ( -1.000000000000000000, 0.000000000000000000, 0.000000000000000000 ) ) ;
#75623=CARTESIAN_POINT ( 'NONE',  ( 191.4749582765727212, 14.19731191252289015, 13.00000000000000178 ) ) ;
#75642=DIRECTION ( 'NONE',  ( -1.000000000000000000, 0.000000000000000000, 0.000000000000000000 ) ) ;
#75671=CARTESIAN_POINT ( 'NONE',  ( 161.2244399300530233, -11.64849832608277325, 13.00000000000000178 ) ) ;
#75803=LINE ( 'NONE', #75345, #80549 ) ;
#76002=EDGE_CURVE ( 'NONE', #14370, #39273, #35006, .T. ) ;
#76195=CIRCLE ( 'NONE', #36863, 4.025000000000000355 ) ;
#76477=ORIENTED_EDGE ( 'NONE', *, *, #16173, .F. ) ;
#76708=ORIENTED_EDGE ( 'NONE', *, *, #12553, .F. ) ;
#77029=DIRECTION ( 'NONE',  ( -0.000000000000000000, -0.000000000000000000, -1.000000000000000000 ) ) ;
#77126=ORIENTED_EDGE ( 'NONE', *, *, #15644, .F. ) ;
#77306=DIRECTION ( 'NONE',  ( -1.000000000000000000, 0.000000000000000000, 0.000000000000000000 ) ) ;
#77637=CARTESIAN_POINT ( 'NONE',  ( 188.7399167944524550, 8.542400036368780647, 13.00000000000000178 ) ) ;
#77707=CARTESIAN_POINT ( 'NONE',  ( 191.4749582765727212, 14.19731191252289015, 13.00000000000000178 ) ) ;
#77785=FACE_OUTER_BOUND ( 'NONE', #81661, .T. ) ;
#77795=DIRECTION ( 'NONE',  ( -1.000000000000000000, 0.000000000000000000, 0.000000000000000000 ) ) ;
#77975=EDGE_CURVE ( 'NONE', #75154, #45901, #21296, .T. ) ;
#78092=DIRECTION ( 'NONE',  ( 1.000000000000000000, 0.000000000000000000, -0.000000000000000000 ) ) ;
#78471=VERTEX_POINT ( 'NONE', #4431 ) ;
#78472=ORIENTED_EDGE ( 'NONE', *, *, #12553, .T. ) ;
#78897=DIRECTION ( 'NONE',  ( -1.000000000000000000, 0.000000000000000000, 0.000000000000000000 ) ) ;
#78922=EDGE_CURVE ( 'NONE', #75154, #35472, #36581, .T. ) ;
#79013=AXIS2_PLACEMENT_3D ( 'NONE', #60063, #24051, #73787 ) ;
#79312=CIRCLE ( 'NONE', #56607, 4.000000000000003553 ) ;
#79924=VERTEX_POINT ( 'NONE', #77707 ) ;
#80483=AXIS2_PLACEMENT_3D ( 'NONE', #17808, #46661, #75565 ) ;
#80542=AXIS2_PLACEMENT_3D ( 'NONE', #83104, #90654, #46649 ) ;
#80549=VECTOR ( 'NONE', #10927, 1000.000000000000000 ) ;
#80688=DIRECTION ( 'NONE',  ( -0.000000000000000000, -0.000000000000000000, -1.000000000000000000 ) ) ;
#81093=ORIENTED_EDGE ( 'NONE', *, *, #41567, .F. ) ;
#81238=ORIENTED_EDGE ( 'NONE', *, *, #15024, .F. ) ;
#81439=SHAPE_REPRESENTATION_RELATIONSHIP ( 'NONE' , 'NONE' ,  #67633, #29498 ) ;
#81571=ORIENTED_EDGE ( 'NONE', *, *, #66872, .T. ) ;
#81661=EDGE_LOOP ( 'NONE', ( #90714, #78472, #61171, #9004 ) ) ;
#82659=FACE_OUTER_BOUND ( 'NONE', #36042, .T. ) ;
#82660=DIRECTION ( 'NONE',  ( -0.000000000000000000, -0.000000000000000000, -1.000000000000000000 ) ) ;
#83104=CARTESIAN_POINT ( 'NONE',  ( 0.000000000000000000, 0.000000000000000000, 10.00000000000000000 ) ) ;
#83253=CARTESIAN_POINT ( 'NONE',  ( 169.2744399300530347, 8.542400036368780647, 13.00000000000000178 ) ) ;
#83433=ADVANCED_FACE ( 'NONE', ( #23554 ), #45768, .F. ) ;
#83518=CIRCLE ( 'NONE', #17031, 4.000000000000003553 ) ;
#83965=EDGE_CURVE ( 'NONE', #45901, #75154, #76195, .T. ) ;
#84136=CARTESIAN_POINT ( 'NONE',  ( 191.4749582765727212, 14.19731191252289015, 10.00000000000000000 ) ) ;
#84629=DIRECTION ( 'NONE',  ( 0.000000000000000000, -0.000000000000000000, -1.000000000000000000 ) ) ;
#84694=DIRECTION ( 'NONE',  ( -0.000000000000000000, -0.000000000000000000, -1.000000000000000000 ) ) ;
#84868=AXIS2_PLACEMENT_3D ( 'NONE', #58926, #80688, #30984 ) ;
#84920=FACE_BOUND ( 'NONE', #72376, .T. ) ;
#85014=VECTOR ( 'NONE', #3609, 1000.000000000000000 ) ;
#85177=DIRECTION ( 'NONE',  ( 1.000000000000000000, 0.000000000000000000, 0.000000000000000000 ) ) ;
#85237=AXIS2_PLACEMENT_3D ( 'NONE', #75623, #11227, #12158 ) ;
#85295=ORIENTED_EDGE ( 'NONE', *, *, #3119, .T. ) ;
#85988=EDGE_LOOP ( 'NONE', ( #64303, #64967, #74614, #29762 ) ) ;
#86848=CIRCLE ( 'NONE', #33939, 4.000000000000003553 ) ;
#87279=EDGE_LOOP ( 'NONE', ( #67578, #2974, #12853, #66853 ) ) ;
#88270=CARTESIAN_POINT ( 'NONE',  ( 165.2494399300530290, -11.64849832608277325, 13.00000000000000178 ) ) ;
#88414=ORIENTED_EDGE ( 'NONE', *, *, #77975, .F. ) ;
#88549=ADVANCED_FACE ( 'NONE', ( #34528 ), #55839, .F. ) ;
#88571=DIRECTION ( 'NONE',  ( 0.000000000000000000, 0.000000000000000000, 1.000000000000000000 ) ) ;
#88676=ADVANCED_FACE ( 'NONE', ( #57256 ), #92739, .F. ) ;
#88734=EDGE_CURVE ( 'NONE', #39273, #59550, #22003, .T. ) ;
#88858=CARTESIAN_POINT ( 'NONE',  ( 165.2494399300530290, -11.64849832608277325, 13.00000000000000178 ) ) ;
#88956=DIRECTION ( 'NONE',  ( -1.000000000000000000, 0.000000000000000000, 0.000000000000000000 ) ) ;
#89206=EDGE_CURVE ( 'NONE', #19058, #25647, #1344, .T. ) ;
#89960=AXIS2_PLACEMENT_3D ( 'NONE', #13234, #78092, #19841 ) ;
#89983=DIRECTION ( 'NONE',  ( 1.000000000000000000, 0.000000000000000000, 0.000000000000000000 ) ) ;
#90079=EDGE_LOOP ( 'NONE', ( #73456, #10162, #18683, #53631 ) ) ;
#90095=AXIS2_PLACEMENT_3D ( 'NONE', #12159, #5545, #78897 ) ;
#90323=LINE ( 'NONE', #75671, #21649 ) ;
#90447=LINE ( 'NONE', #68716, #23029 ) ;
#90654=DIRECTION ( 'NONE',  ( -0.000000000000000000, 0.000000000000000000, -1.000000000000000000 ) ) ;
#90714=ORIENTED_EDGE ( 'NONE', *, *, #71361, .F. ) ;
#90725=PLANE ( 'NONE',  #85237 ) ;
#90791=CARTESIAN_POINT ( 'NONE',  ( 184.7149167944524493, -12.49482340714361506, 13.00000000000000178 ) ) ;
#90959=CARTESIAN_POINT ( 'NONE',  ( 0.000000000000000000, 0.000000000000000000, 0.000000000000000000 ) ) ;
#91002=DIRECTION ( 'NONE',  ( -0.000000000000000000, -0.000000000000000000, -1.000000000000000000 ) ) ;
#91229=VECTOR ( 'NONE', #19436, 1000.000000000000000 ) ;
#91573=EDGE_CURVE ( 'NONE', #59550, #39273, #28163, .T. ) ;
#92065=PRODUCT_DEFINITION_CONTEXT ( 'detailed design', #17230, 'design' ) ;
#92488=DIRECTION ( 'NONE',  ( -1.000000000000000000, 0.000000000000000000, 0.000000000000000000 ) ) ;
#92739=PLANE ( 'NONE',  #89960 ) ;
#93028=ADVANCED_FACE ( 'NONE', ( #6471 ), #6003, .F. ) ;
#93705=VERTEX_POINT ( 'NONE', #39846 ) ;
#93732=COLOUR_RGB('Light Blue',0.38,0.62,0.78);
#93733=FILL_AREA_STYLE_COLOUR('',#93732);
#93734=FILL_AREA_STYLE('',(#93733));
#93735=SURFACE_STYLE_FILL_AREA(#93734);
#93736=SURFACE_SIDE_STYLE('',(#93735));
#93737=SURFACE_STYLE_USAGE(.BOTH.,#93736);
#93738=PRESENTATION_STYLE_ASSIGNMENT((#93737));
ENDSEC;
END-ISO-10303-21;
